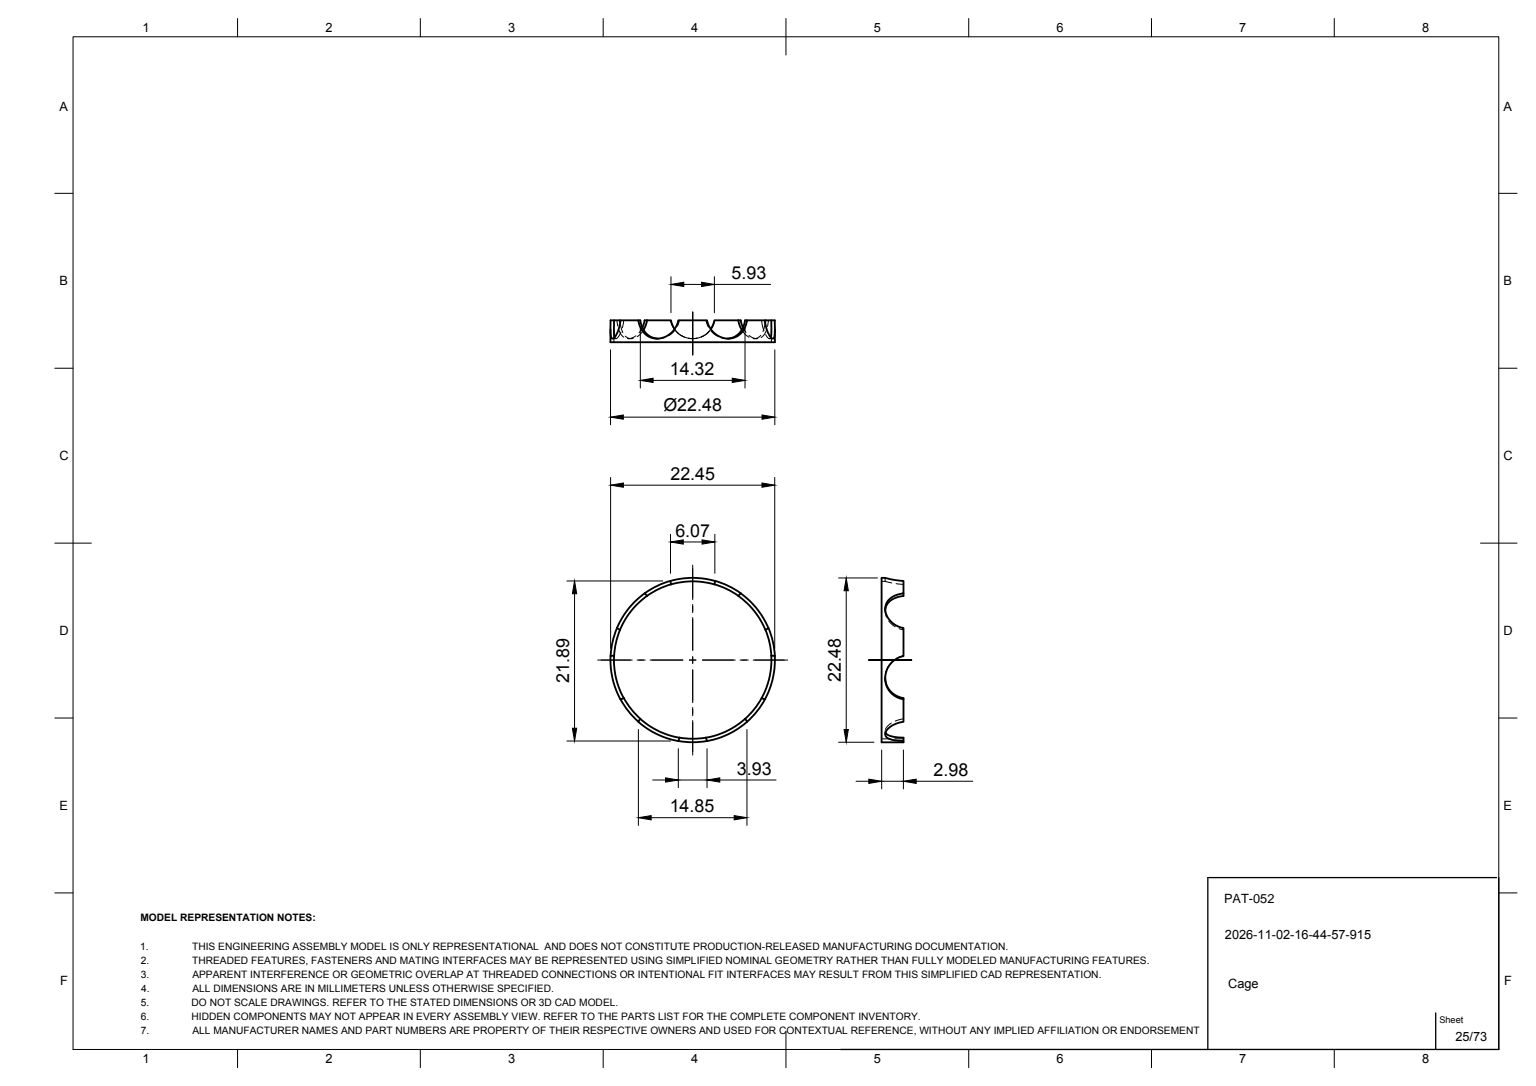
ISO-10303-21;
HEADER;
/* Generated by software containing ST-Developer
 * from STEP Tools, Inc. (www.steptools.com) 
 */

FILE_DESCRIPTION(
/* description */ ('Hand-crank gear train demonstrator'),
/* implementation_level */ '2;1');

FILE_NAME(
/* name */ 'Cage.step',
/* time_stamp */ '2026-10-28T03:22:13-07:00',
/* author */ (''),
/* organization */ (''),
/* preprocessor_version */ 'ST-DEVELOPER v20.2',
/* originating_system */ 'Autodesk Translation Framework v15.17.0.0',
/* authorisation */ '');

FILE_SCHEMA (('AUTOMOTIVE_DESIGN { 1 0 10303 214 3 1 1 }'));
ENDSEC;

DATA;
#10=MECHANICAL_DESIGN_GEOMETRIC_PRESENTATION_REPRESENTATION('',(#1209),#62758);
#859=B_SPLINE_CURVE_WITH_KNOTS('',3,(#24083,#24084,#24085,#24086,#24087,
#24088,#24089,#24090,#24091,#24092,#24093,#24094,#24095,#24096,#24097,#24098,
#24099,#24100,#24101,#24102,#24103,#24104),.UNSPECIFIED.,.F.,.F.,(4,2,2,
2,2,2,2,2,2,2,4),(0.0591825211272536,0.157966726598481,0.236950089897721,
0.315933453196962,0.391576304923761,0.46721915665056,0.54286200837736,0.618504860104159,
0.697488223403399,0.77647158670264,0.875255792173867),.UNSPECIFIED.);
#860=B_SPLINE_CURVE_WITH_KNOTS('',3,(#24108,#24109,#24110,#24111,#24112,
#24113,#24114,#24115,#24116,#24117,#24118,#24119,#24120,#24121,#24122,#24123,
#24124,#24125,#24126,#24127,#24128,#24129),.UNSPECIFIED.,.F.,.F.,(4,2,2,
2,2,2,2,2,2,2,4),(0.0581119756758434,0.106553146291161,0.213106292582322,
0.30849933801665,0.386091982889075,0.4636846277615,0.541277272633925,0.61886991750635,
0.714262962940678,0.820816109231839,0.869257279847157),.UNSPECIFIED.);
#861=B_SPLINE_CURVE_WITH_KNOTS('',3,(#24135,#24136,#24137,#24138,#24139,
#24140,#24141,#24142,#24143,#24144,#24145,#24146,#24147,#24148,#24149,#24150,
#24151,#24152,#24153,#24154,#24155,#24156),.UNSPECIFIED.,.F.,.F.,(4,2,2,
2,2,2,2,2,2,2,4),(0.0581119756758434,0.106553146291161,0.213106292582322,
0.30849933801665,0.386091982889075,0.4636846277615,0.541277272633925,0.61886991750635,
0.714262962940679,0.820816109231839,0.869257279847157),.UNSPECIFIED.);
#862=B_SPLINE_CURVE_WITH_KNOTS('',3,(#24160,#24161,#24162,#24163,#24164,
#24165,#24166,#24167,#24168,#24169,#24170,#24171,#24172,#24173,#24174,#24175,
#24176,#24177,#24178,#24179,#24180,#24181),.UNSPECIFIED.,.F.,.F.,(4,2,2,
2,2,2,2,2,2,2,4),(0.0581119756758433,0.106553146291161,0.213106292582322,
0.308499338016649,0.386091982889075,0.4636846277615,0.541277272633925,0.61886991750635,
0.714262962940678,0.820816109231839,0.869257279847157),.UNSPECIFIED.);
#863=B_SPLINE_CURVE_WITH_KNOTS('',3,(#24190,#24191,#24192,#24193,#24194,
#24195,#24196,#24197,#24198,#24199,#24200,#24201,#24202,#24203,#24204,#24205,
#24206,#24207,#24208,#24209,#24210,#24211),.UNSPECIFIED.,.F.,.F.,(4,2,2,
2,2,2,2,2,2,2,4),(0.0581119756758433,0.106553146291161,0.213106292582322,
0.30849933801665,0.386091982889075,0.4636846277615,0.541277272633925,0.61886991750635,
0.714262962940678,0.820816109231839,0.869257279847157),.UNSPECIFIED.);
#864=B_SPLINE_CURVE_WITH_KNOTS('',3,(#24215,#24216,#24217,#24218,#24219,
#24220,#24221,#24222,#24223,#24224,#24225,#24226,#24227,#24228,#24229,#24230,
#24231,#24232,#24233,#24234,#24235,#24236),.UNSPECIFIED.,.F.,.F.,(4,2,2,
2,2,2,2,2,2,2,4),(0.0581119756758434,0.106553146291161,0.213106292582322,
0.30849933801665,0.386091982889075,0.4636846277615,0.541277272633925,0.61886991750635,
0.714262962940678,0.820816109231839,0.869257279847157),.UNSPECIFIED.);
#865=B_SPLINE_CURVE_WITH_KNOTS('',3,(#24240,#24241,#24242,#24243,#24244,
#24245,#24246,#24247,#24248,#24249,#24250,#24251,#24252,#24253,#24254,#24255,
#24256,#24257,#24258,#24259,#24260,#24261),.UNSPECIFIED.,.F.,.F.,(4,2,2,
2,2,2,2,2,2,2,4),(0.0581119756758434,0.106553146291161,0.213106292582322,
0.30849933801665,0.386091982889075,0.4636846277615,0.541277272633925,0.61886991750635,
0.714262962940678,0.820816109231839,0.869257279847157),.UNSPECIFIED.);
#866=B_SPLINE_CURVE_WITH_KNOTS('',3,(#24265,#24266,#24267,#24268,#24269,
#24270,#24271,#24272,#24273,#24274,#24275,#24276,#24277,#24278,#24279,#24280,
#24281,#24282,#24283,#24284,#24285,#24286),.UNSPECIFIED.,.F.,.F.,(4,2,2,
2,2,2,2,2,2,2,4),(0.0581119756758433,0.106553146291161,0.213106292582322,
0.30849933801665,0.386091982889075,0.4636846277615,0.541277272633925,0.61886991750635,
0.714262962940678,0.820816109231839,0.869257279847157),.UNSPECIFIED.);
#867=B_SPLINE_CURVE_WITH_KNOTS('',3,(#24294,#24295,#24296,#24297,#24298,
#24299,#24300,#24301,#24302,#24303,#24304,#24305,#24306,#24307,#24308,#24309,
#24310,#24311,#24312,#24313,#24314,#24315),.UNSPECIFIED.,.F.,.F.,(4,2,2,
2,2,2,2,2,2,2,4),(0.0591825211272536,0.157966726598481,0.236950089897721,
0.315933453196962,0.391576304923761,0.467219156650561,0.54286200837736,
0.618504860104159,0.697488223403399,0.77647158670264,0.875255792173867),
 .UNSPECIFIED.);
#868=B_SPLINE_CURVE_WITH_KNOTS('',3,(#24323,#24324,#24325,#24326,#24327,
#24328,#24329,#24330,#24331,#24332,#24333,#24334,#24335,#24336,#24337,#24338,
#24339,#24340,#24341,#24342,#24343,#24344),.UNSPECIFIED.,.F.,.F.,(4,2,2,
2,2,2,2,2,2,2,4),(0.0591825211272536,0.157966726598481,0.236950089897722,
0.315933453196962,0.391576304923761,0.467219156650561,0.54286200837736,
0.618504860104159,0.697488223403399,0.77647158670264,0.875255792173867),
 .UNSPECIFIED.);
#869=B_SPLINE_CURVE_WITH_KNOTS('',3,(#24354,#24355,#24356,#24357,#24358,
#24359,#24360,#24361,#24362,#24363,#24364,#24365,#24366,#24367,#24368,#24369,
#24370,#24371,#24372,#24373,#24374,#24375),.UNSPECIFIED.,.F.,.F.,(4,2,2,
2,2,2,2,2,2,2,4),(0.0591825211272536,0.157966726598481,0.236950089897721,
0.315933453196962,0.391576304923761,0.46721915665056,0.54286200837736,0.618504860104159,
0.697488223403399,0.77647158670264,0.875255792173867),.UNSPECIFIED.);
#870=B_SPLINE_CURVE_WITH_KNOTS('',3,(#24383,#24384,#24385,#24386,#24387,
#24388,#24389,#24390,#24391,#24392,#24393,#24394,#24395,#24396,#24397,#24398,
#24399,#24400,#24401,#24402,#24403,#24404),.UNSPECIFIED.,.F.,.F.,(4,2,2,
2,2,2,2,2,2,2,4),(0.0591825211272536,0.157966726598481,0.236950089897721,
0.315933453196962,0.391576304923761,0.46721915665056,0.542862008377359,
0.618504860104159,0.697488223403399,0.776471586702639,0.875255792173867),
 .UNSPECIFIED.);
#871=B_SPLINE_CURVE_WITH_KNOTS('',3,(#24412,#24413,#24414,#24415,#24416,
#24417,#24418,#24419,#24420,#24421,#24422,#24423,#24424,#24425,#24426,#24427,
#24428,#24429,#24430,#24431,#24432,#24433),.UNSPECIFIED.,.F.,.F.,(4,2,2,
2,2,2,2,2,2,2,4),(0.0591825211272536,0.157966726598481,0.236950089897721,
0.315933453196962,0.391576304923761,0.46721915665056,0.54286200837736,0.618504860104159,
0.697488223403399,0.77647158670264,0.875255792173867),.UNSPECIFIED.);
#872=B_SPLINE_CURVE_WITH_KNOTS('',3,(#24442,#24443,#24444,#24445,#24446,
#24447,#24448,#24449,#24450,#24451,#24452,#24453,#24454,#24455,#24456,#24457,
#24458,#24459,#24460,#24461,#24462,#24463),.UNSPECIFIED.,.F.,.F.,(4,2,2,
2,2,2,2,2,2,2,4),(0.0591825211272536,0.157966726598481,0.236950089897721,
0.315933453196962,0.391576304923761,0.46721915665056,0.542862008377359,
0.618504860104159,0.697488223403399,0.776471586702639,0.875255792173867),
 .UNSPECIFIED.);
#998=SPHERICAL_SURFACE('',#17541,0.309556);
#999=SPHERICAL_SURFACE('',#17557,0.309556);
#1000=SPHERICAL_SURFACE('',#17562,0.309556);
#1001=SPHERICAL_SURFACE('',#17568,0.309556);
#1002=SPHERICAL_SURFACE('',#17573,0.309556);
#1003=SPHERICAL_SURFACE('',#17578,0.309556);
#1004=SPHERICAL_SURFACE('',#17586,0.309556);
#1075=SHAPE_REPRESENTATION_RELATIONSHIP('SRR','None',#63048,#1139);
#1139=ADVANCED_BREP_SHAPE_REPRESENTATION('',(#1287),#62702);
#1209=STYLED_ITEM('',(#63462),#1287);
#1287=MANIFOLD_SOLID_BREP('Continuous crown cage',#16390);
#1491=FACE_BOUND('',#3385,.T.);
#1686=PLANE('',#17554);
#1687=PLANE('',#17559);
#1688=PLANE('',#17564);
#1689=PLANE('',#17570);
#1690=PLANE('',#17575);
#1691=PLANE('',#17584);
#1692=PLANE('',#17588);
#1693=PLANE('',#17589);
#2284=FACE_OUTER_BOUND('',#3369,.T.);
#2285=FACE_OUTER_BOUND('',#3370,.T.);
#2286=FACE_OUTER_BOUND('',#3371,.T.);
#2287=FACE_OUTER_BOUND('',#3372,.T.);
#2288=FACE_OUTER_BOUND('',#3373,.T.);
#2289=FACE_OUTER_BOUND('',#3374,.T.);
#2290=FACE_OUTER_BOUND('',#3375,.T.);
#2291=FACE_OUTER_BOUND('',#3376,.T.);
#2292=FACE_OUTER_BOUND('',#3377,.T.);
#2293=FACE_OUTER_BOUND('',#3378,.T.);
#2294=FACE_OUTER_BOUND('',#3379,.T.);
#2295=FACE_OUTER_BOUND('',#3380,.T.);
#2296=FACE_OUTER_BOUND('',#3381,.T.);
#2297=FACE_OUTER_BOUND('',#3382,.T.);
#2298=FACE_OUTER_BOUND('',#3383,.T.);
#2299=FACE_OUTER_BOUND('',#3384,.T.);
#2300=FACE_OUTER_BOUND('',#3386,.T.);
#3369=EDGE_LOOP('',(#11537,#11538,#11539,#11540));
#3370=EDGE_LOOP('',(#11541,#11542,#11543,#11544,#11545,#11546,#11547,#11548,
#11549,#11550,#11551,#11552,#11553,#11554,#11555,#11556,#11557,#11558));
#3371=EDGE_LOOP('',(#11559,#11560,#11561,#11562));
#3372=EDGE_LOOP('',(#11563,#11564,#11565,#11566));
#3373=EDGE_LOOP('',(#11567,#11568,#11569,#11570));
#3374=EDGE_LOOP('',(#11571,#11572,#11573,#11574));
#3375=EDGE_LOOP('',(#11575,#11576,#11577,#11578,#11579,#11580));
#3376=EDGE_LOOP('',(#11581,#11582,#11583,#11584));
#3377=EDGE_LOOP('',(#11585,#11586,#11587,#11588));
#3378=EDGE_LOOP('',(#11589,#11590,#11591,#11592));
#3379=EDGE_LOOP('',(#11593,#11594,#11595,#11596));
#3380=EDGE_LOOP('',(#11597,#11598,#11599,#11600));
#3381=EDGE_LOOP('',(#11601,#11602,#11603,#11604,#11605,#11606,#11607,#11608,
#11609,#11610,#11611,#11612,#11613,#11614,#11615,#11616,#11617,#11618));
#3382=EDGE_LOOP('',(#11619,#11620,#11621,#11622));
#3383=EDGE_LOOP('',(#11623,#11624,#11625,#11626));
#3384=EDGE_LOOP('',(#11627));
#3385=EDGE_LOOP('',(#11628));
#3386=EDGE_LOOP('',(#11629,#11630,#11631,#11632));
#4433=LINE('',#24185,#5565);
#4434=LINE('',#24438,#5566);
#5565=VECTOR('',#19758,1.123812);
#5566=VECTOR('',#19827,1.076188);
#6754=CIRCLE('',#17542,0.303778037777585);
#6755=CIRCLE('',#17543,0.303778037777585);
#6756=CIRCLE('',#17545,1.123812);
#6757=CIRCLE('',#17546,1.123812);
#6758=CIRCLE('',#17547,1.123812);
#6759=CIRCLE('',#17548,1.123812);
#6760=CIRCLE('',#17549,1.123812);
#6761=CIRCLE('',#17550,1.123812);
#6762=CIRCLE('',#17551,1.123812);
#6763=CIRCLE('',#17552,1.123812);
#6764=CIRCLE('',#17553,1.123812);
#6765=CIRCLE('',#17555,1.076188);
#6766=CIRCLE('',#17556,0.303778037777585);
#6767=CIRCLE('',#17558,0.303778037777585);
#6768=CIRCLE('',#17560,1.076188);
#6769=CIRCLE('',#17561,0.303778037777585);
#6770=CIRCLE('',#17563,0.303778037777585);
#6771=CIRCLE('',#17565,1.076188);
#6772=CIRCLE('',#17566,1.076188);
#6773=CIRCLE('',#17567,0.303778037777585);
#6774=CIRCLE('',#17569,0.303778037777585);
#6775=CIRCLE('',#17571,1.076188);
#6776=CIRCLE('',#17572,0.303778037777585);
#6777=CIRCLE('',#17574,0.303778037777585);
#6778=CIRCLE('',#17576,1.076188);
#6779=CIRCLE('',#17577,0.303778037777585);
#6780=CIRCLE('',#17579,0.303778037777585);
#6781=CIRCLE('',#17581,1.076188);
#6782=CIRCLE('',#17582,1.076188);
#6783=CIRCLE('',#17583,1.076188);
#6784=CIRCLE('',#17585,0.303778037777585);
#6785=CIRCLE('',#17587,0.303778037777585);
#7453=VERTEX_POINT('',#24081);
#7454=VERTEX_POINT('',#24082);
#7455=VERTEX_POINT('',#24105);
#7456=VERTEX_POINT('',#24107);
#7457=VERTEX_POINT('',#24132);
#7458=VERTEX_POINT('',#24134);
#7459=VERTEX_POINT('',#24157);
#7460=VERTEX_POINT('',#24159);
#7461=VERTEX_POINT('',#24182);
#7462=VERTEX_POINT('',#24184);
#7463=VERTEX_POINT('',#24187);
#7464=VERTEX_POINT('',#24189);
#7465=VERTEX_POINT('',#24212);
#7466=VERTEX_POINT('',#24214);
#7467=VERTEX_POINT('',#24237);
#7468=VERTEX_POINT('',#24239);
#7469=VERTEX_POINT('',#24262);
#7470=VERTEX_POINT('',#24264);
#7471=VERTEX_POINT('',#24289);
#7472=VERTEX_POINT('',#24293);
#7473=VERTEX_POINT('',#24318);
#7474=VERTEX_POINT('',#24322);
#7475=VERTEX_POINT('',#24347);
#7476=VERTEX_POINT('',#24349);
#7477=VERTEX_POINT('',#24353);
#7478=VERTEX_POINT('',#24378);
#7479=VERTEX_POINT('',#24382);
#7480=VERTEX_POINT('',#24407);
#7481=VERTEX_POINT('',#24411);
#7482=VERTEX_POINT('',#24436);
#7483=VERTEX_POINT('',#24439);
#7484=VERTEX_POINT('',#24441);
#9020=EDGE_CURVE('',#7453,#7454,#859,.T.);
#9021=EDGE_CURVE('',#7455,#7453,#6754,.T.);
#9022=EDGE_CURVE('',#7456,#7455,#860,.T.);
#9023=EDGE_CURVE('',#7454,#7456,#6755,.T.);
#9024=EDGE_CURVE('',#7457,#7455,#6756,.T.);
#9025=EDGE_CURVE('',#7457,#7458,#861,.T.);
#9026=EDGE_CURVE('',#7459,#7458,#6757,.T.);
#9027=EDGE_CURVE('',#7459,#7460,#862,.T.);
#9028=EDGE_CURVE('',#7461,#7460,#6758,.T.);
#9029=EDGE_CURVE('',#7461,#7462,#4433,.T.);
#9030=EDGE_CURVE('',#7462,#7462,#6759,.T.);
#9031=EDGE_CURVE('',#7463,#7461,#6760,.T.);
#9032=EDGE_CURVE('',#7463,#7464,#863,.T.);
#9033=EDGE_CURVE('',#7465,#7464,#6761,.T.);
#9034=EDGE_CURVE('',#7465,#7466,#864,.T.);
#9035=EDGE_CURVE('',#7467,#7466,#6762,.T.);
#9036=EDGE_CURVE('',#7467,#7468,#865,.T.);
#9037=EDGE_CURVE('',#7469,#7468,#6763,.T.);
#9038=EDGE_CURVE('',#7469,#7470,#866,.T.);
#9039=EDGE_CURVE('',#7456,#7470,#6764,.T.);
#9040=EDGE_CURVE('',#7453,#7471,#6765,.T.);
#9041=EDGE_CURVE('',#7471,#7457,#6766,.T.);
#9042=EDGE_CURVE('',#7472,#7471,#867,.T.);
#9043=EDGE_CURVE('',#7458,#7472,#6767,.T.);
#9044=EDGE_CURVE('',#7472,#7473,#6768,.T.);
#9045=EDGE_CURVE('',#7473,#7459,#6769,.T.);
#9046=EDGE_CURVE('',#7474,#7473,#868,.T.);
#9047=EDGE_CURVE('',#7460,#7474,#6770,.T.);
#9048=EDGE_CURVE('',#7474,#7475,#6771,.T.);
#9049=EDGE_CURVE('',#7475,#7476,#6772,.T.);
#9050=EDGE_CURVE('',#7476,#7463,#6773,.T.);
#9051=EDGE_CURVE('',#7477,#7476,#869,.T.);
#9052=EDGE_CURVE('',#7464,#7477,#6774,.T.);
#9053=EDGE_CURVE('',#7477,#7478,#6775,.T.);
#9054=EDGE_CURVE('',#7478,#7465,#6776,.T.);
#9055=EDGE_CURVE('',#7479,#7478,#870,.T.);
#9056=EDGE_CURVE('',#7466,#7479,#6777,.T.);
#9057=EDGE_CURVE('',#7479,#7480,#6778,.T.);
#9058=EDGE_CURVE('',#7480,#7467,#6779,.T.);
#9059=EDGE_CURVE('',#7481,#7480,#871,.T.);
#9060=EDGE_CURVE('',#7468,#7481,#6780,.T.);
#9061=EDGE_CURVE('',#7482,#7482,#6781,.T.);
#9062=EDGE_CURVE('',#7482,#7475,#4434,.T.);
#9063=EDGE_CURVE('',#7483,#7454,#6782,.T.);
#9064=EDGE_CURVE('',#7483,#7484,#872,.T.);
#9065=EDGE_CURVE('',#7481,#7484,#6783,.T.);
#9066=EDGE_CURVE('',#7470,#7483,#6784,.T.);
#9067=EDGE_CURVE('',#7484,#7469,#6785,.T.);
#11537=ORIENTED_EDGE('',*,*,#9020,.F.);
#11538=ORIENTED_EDGE('',*,*,#9021,.F.);
#11539=ORIENTED_EDGE('',*,*,#9022,.F.);
#11540=ORIENTED_EDGE('',*,*,#9023,.F.);
#11541=ORIENTED_EDGE('',*,*,#9022,.T.);
#11542=ORIENTED_EDGE('',*,*,#9024,.F.);
#11543=ORIENTED_EDGE('',*,*,#9025,.T.);
#11544=ORIENTED_EDGE('',*,*,#9026,.F.);
#11545=ORIENTED_EDGE('',*,*,#9027,.T.);
#11546=ORIENTED_EDGE('',*,*,#9028,.F.);
#11547=ORIENTED_EDGE('',*,*,#9029,.T.);
#11548=ORIENTED_EDGE('',*,*,#9030,.F.);
#11549=ORIENTED_EDGE('',*,*,#9029,.F.);
#11550=ORIENTED_EDGE('',*,*,#9031,.F.);
#11551=ORIENTED_EDGE('',*,*,#9032,.T.);
#11552=ORIENTED_EDGE('',*,*,#9033,.F.);
#11553=ORIENTED_EDGE('',*,*,#9034,.T.);
#11554=ORIENTED_EDGE('',*,*,#9035,.F.);
#11555=ORIENTED_EDGE('',*,*,#9036,.T.);
#11556=ORIENTED_EDGE('',*,*,#9037,.F.);
#11557=ORIENTED_EDGE('',*,*,#9038,.T.);
#11558=ORIENTED_EDGE('',*,*,#9039,.F.);
#11559=ORIENTED_EDGE('',*,*,#9021,.T.);
#11560=ORIENTED_EDGE('',*,*,#9040,.T.);
#11561=ORIENTED_EDGE('',*,*,#9041,.T.);
#11562=ORIENTED_EDGE('',*,*,#9024,.T.);
#11563=ORIENTED_EDGE('',*,*,#9042,.F.);
#11564=ORIENTED_EDGE('',*,*,#9043,.F.);
#11565=ORIENTED_EDGE('',*,*,#9025,.F.);
#11566=ORIENTED_EDGE('',*,*,#9041,.F.);
#11567=ORIENTED_EDGE('',*,*,#9043,.T.);
#11568=ORIENTED_EDGE('',*,*,#9044,.T.);
#11569=ORIENTED_EDGE('',*,*,#9045,.T.);
#11570=ORIENTED_EDGE('',*,*,#9026,.T.);
#11571=ORIENTED_EDGE('',*,*,#9046,.F.);
#11572=ORIENTED_EDGE('',*,*,#9047,.F.);
#11573=ORIENTED_EDGE('',*,*,#9027,.F.);
#11574=ORIENTED_EDGE('',*,*,#9045,.F.);
#11575=ORIENTED_EDGE('',*,*,#9047,.T.);
#11576=ORIENTED_EDGE('',*,*,#9048,.T.);
#11577=ORIENTED_EDGE('',*,*,#9049,.T.);
#11578=ORIENTED_EDGE('',*,*,#9050,.T.);
#11579=ORIENTED_EDGE('',*,*,#9031,.T.);
#11580=ORIENTED_EDGE('',*,*,#9028,.T.);
#11581=ORIENTED_EDGE('',*,*,#9051,.F.);
#11582=ORIENTED_EDGE('',*,*,#9052,.F.);
#11583=ORIENTED_EDGE('',*,*,#9032,.F.);
#11584=ORIENTED_EDGE('',*,*,#9050,.F.);
#11585=ORIENTED_EDGE('',*,*,#9052,.T.);
#11586=ORIENTED_EDGE('',*,*,#9053,.T.);
#11587=ORIENTED_EDGE('',*,*,#9054,.T.);
#11588=ORIENTED_EDGE('',*,*,#9033,.T.);
#11589=ORIENTED_EDGE('',*,*,#9055,.F.);
#11590=ORIENTED_EDGE('',*,*,#9056,.F.);
#11591=ORIENTED_EDGE('',*,*,#9034,.F.);
#11592=ORIENTED_EDGE('',*,*,#9054,.F.);
#11593=ORIENTED_EDGE('',*,*,#9056,.T.);
#11594=ORIENTED_EDGE('',*,*,#9057,.T.);
#11595=ORIENTED_EDGE('',*,*,#9058,.T.);
#11596=ORIENTED_EDGE('',*,*,#9035,.T.);
#11597=ORIENTED_EDGE('',*,*,#9036,.F.);
#11598=ORIENTED_EDGE('',*,*,#9058,.F.);
#11599=ORIENTED_EDGE('',*,*,#9059,.F.);
#11600=ORIENTED_EDGE('',*,*,#9060,.F.);
#11601=ORIENTED_EDGE('',*,*,#9061,.F.);
#11602=ORIENTED_EDGE('',*,*,#9062,.T.);
#11603=ORIENTED_EDGE('',*,*,#9048,.F.);
#11604=ORIENTED_EDGE('',*,*,#9046,.T.);
#11605=ORIENTED_EDGE('',*,*,#9044,.F.);
#11606=ORIENTED_EDGE('',*,*,#9042,.T.);
#11607=ORIENTED_EDGE('',*,*,#9040,.F.);
#11608=ORIENTED_EDGE('',*,*,#9020,.T.);
#11609=ORIENTED_EDGE('',*,*,#9063,.F.);
#11610=ORIENTED_EDGE('',*,*,#9064,.T.);
#11611=ORIENTED_EDGE('',*,*,#9065,.F.);
#11612=ORIENTED_EDGE('',*,*,#9059,.T.);
#11613=ORIENTED_EDGE('',*,*,#9057,.F.);
#11614=ORIENTED_EDGE('',*,*,#9055,.T.);
#11615=ORIENTED_EDGE('',*,*,#9053,.F.);
#11616=ORIENTED_EDGE('',*,*,#9051,.T.);
#11617=ORIENTED_EDGE('',*,*,#9049,.F.);
#11618=ORIENTED_EDGE('',*,*,#9062,.F.);
#11619=ORIENTED_EDGE('',*,*,#9023,.T.);
#11620=ORIENTED_EDGE('',*,*,#9039,.T.);
#11621=ORIENTED_EDGE('',*,*,#9066,.T.);
#11622=ORIENTED_EDGE('',*,*,#9063,.T.);
#11623=ORIENTED_EDGE('',*,*,#9038,.F.);
#11624=ORIENTED_EDGE('',*,*,#9067,.F.);
#11625=ORIENTED_EDGE('',*,*,#9064,.F.);
#11626=ORIENTED_EDGE('',*,*,#9066,.F.);
#11627=ORIENTED_EDGE('',*,*,#9030,.T.);
#11628=ORIENTED_EDGE('',*,*,#9061,.T.);
#11629=ORIENTED_EDGE('',*,*,#9060,.T.);
#11630=ORIENTED_EDGE('',*,*,#9065,.T.);
#11631=ORIENTED_EDGE('',*,*,#9067,.T.);
#11632=ORIENTED_EDGE('',*,*,#9037,.T.);
#15259=CYLINDRICAL_SURFACE('',#17544,1.123812);
#15260=CYLINDRICAL_SURFACE('',#17580,1.076188);
#15594=ADVANCED_FACE('',(#2284),#998,.F.);
#15595=ADVANCED_FACE('',(#2285),#15259,.T.);
#15596=ADVANCED_FACE('',(#2286),#1686,.T.);
#15597=ADVANCED_FACE('',(#2287),#999,.F.);
#15598=ADVANCED_FACE('',(#2288),#1687,.T.);
#15599=ADVANCED_FACE('',(#2289),#1000,.F.);
#15600=ADVANCED_FACE('',(#2290),#1688,.T.);
#15601=ADVANCED_FACE('',(#2291),#1001,.F.);
#15602=ADVANCED_FACE('',(#2292),#1689,.T.);
#15603=ADVANCED_FACE('',(#2293),#1002,.F.);
#15604=ADVANCED_FACE('',(#2294),#1690,.T.);
#15605=ADVANCED_FACE('',(#2295),#1003,.F.);
#15606=ADVANCED_FACE('',(#2296),#15260,.F.);
#15607=ADVANCED_FACE('',(#2297),#1691,.T.);
#15608=ADVANCED_FACE('',(#2298),#1004,.F.);
#15609=ADVANCED_FACE('',(#2299,#1491),#1692,.T.);
#15610=ADVANCED_FACE('',(#2300),#1693,.T.);
#16390=CLOSED_SHELL('',(#15594,#15595,#15596,#15597,#15598,#15599,#15600,
#15601,#15602,#15603,#15604,#15605,#15606,#15607,#15608,#15609,#15610));
#17540=AXIS2_PLACEMENT_3D('',#24079,#19742,#19743);
#17541=AXIS2_PLACEMENT_3D('',#24080,#19744,#19745);
#17542=AXIS2_PLACEMENT_3D('',#24106,#19746,#19747);
#17543=AXIS2_PLACEMENT_3D('',#24130,#19748,#19749);
#17544=AXIS2_PLACEMENT_3D('',#24131,#19750,#19751);
#17545=AXIS2_PLACEMENT_3D('',#24133,#19752,#19753);
#17546=AXIS2_PLACEMENT_3D('',#24158,#19754,#19755);
#17547=AXIS2_PLACEMENT_3D('',#24183,#19756,#19757);
#17548=AXIS2_PLACEMENT_3D('',#24186,#19759,#19760);
#17549=AXIS2_PLACEMENT_3D('',#24188,#19761,#19762);
#17550=AXIS2_PLACEMENT_3D('',#24213,#19763,#19764);
#17551=AXIS2_PLACEMENT_3D('',#24238,#19765,#19766);
#17552=AXIS2_PLACEMENT_3D('',#24263,#19767,#19768);
#17553=AXIS2_PLACEMENT_3D('',#24287,#19769,#19770);
#17554=AXIS2_PLACEMENT_3D('',#24288,#19771,#19772);
#17555=AXIS2_PLACEMENT_3D('',#24290,#19773,#19774);
#17556=AXIS2_PLACEMENT_3D('',#24291,#19775,#19776);
#17557=AXIS2_PLACEMENT_3D('',#24292,#19777,#19778);
#17558=AXIS2_PLACEMENT_3D('',#24316,#19779,#19780);
#17559=AXIS2_PLACEMENT_3D('',#24317,#19781,#19782);
#17560=AXIS2_PLACEMENT_3D('',#24319,#19783,#19784);
#17561=AXIS2_PLACEMENT_3D('',#24320,#19785,#19786);
#17562=AXIS2_PLACEMENT_3D('',#24321,#19787,#19788);
#17563=AXIS2_PLACEMENT_3D('',#24345,#19789,#19790);
#17564=AXIS2_PLACEMENT_3D('',#24346,#19791,#19792);
#17565=AXIS2_PLACEMENT_3D('',#24348,#19793,#19794);
#17566=AXIS2_PLACEMENT_3D('',#24350,#19795,#19796);
#17567=AXIS2_PLACEMENT_3D('',#24351,#19797,#19798);
#17568=AXIS2_PLACEMENT_3D('',#24352,#19799,#19800);
#17569=AXIS2_PLACEMENT_3D('',#24376,#19801,#19802);
#17570=AXIS2_PLACEMENT_3D('',#24377,#19803,#19804);
#17571=AXIS2_PLACEMENT_3D('',#24379,#19805,#19806);
#17572=AXIS2_PLACEMENT_3D('',#24380,#19807,#19808);
#17573=AXIS2_PLACEMENT_3D('',#24381,#19809,#19810);
#17574=AXIS2_PLACEMENT_3D('',#24405,#19811,#19812);
#17575=AXIS2_PLACEMENT_3D('',#24406,#19813,#19814);
#17576=AXIS2_PLACEMENT_3D('',#24408,#19815,#19816);
#17577=AXIS2_PLACEMENT_3D('',#24409,#19817,#19818);
#17578=AXIS2_PLACEMENT_3D('',#24410,#19819,#19820);
#17579=AXIS2_PLACEMENT_3D('',#24434,#19821,#19822);
#17580=AXIS2_PLACEMENT_3D('',#24435,#19823,#19824);
#17581=AXIS2_PLACEMENT_3D('',#24437,#19825,#19826);
#17582=AXIS2_PLACEMENT_3D('',#24440,#19828,#19829);
#17583=AXIS2_PLACEMENT_3D('',#24464,#19830,#19831);
#17584=AXIS2_PLACEMENT_3D('',#24465,#19832,#19833);
#17585=AXIS2_PLACEMENT_3D('',#24466,#19834,#19835);
#17586=AXIS2_PLACEMENT_3D('',#24467,#19836,#19837);
#17587=AXIS2_PLACEMENT_3D('',#24468,#19838,#19839);
#17588=AXIS2_PLACEMENT_3D('',#24469,#19840,#19841);
#17589=AXIS2_PLACEMENT_3D('',#24470,#19842,#19843);
#19742=DIRECTION('axis',(0.,0.,1.));
#19743=DIRECTION('refdir',(1.,0.,0.));
#19744=DIRECTION('center_axis',(0.,0.,1.));
#19745=DIRECTION('ref_axis',(1.,0.,0.));
#19746=DIRECTION('center_axis',(0.,-1.,0.));
#19747=DIRECTION('ref_axis',(0.,0.,-1.));
#19748=DIRECTION('center_axis',(0.,-1.,0.));
#19749=DIRECTION('ref_axis',(0.,0.,-1.));
#19750=DIRECTION('center_axis',(0.,1.,0.));
#19751=DIRECTION('ref_axis',(1.,0.,0.));
#19752=DIRECTION('center_axis',(0.,1.,0.));
#19753=DIRECTION('ref_axis',(1.,0.,0.));
#19754=DIRECTION('center_axis',(0.,1.,0.));
#19755=DIRECTION('ref_axis',(1.,0.,0.));
#19756=DIRECTION('center_axis',(0.,1.,0.));
#19757=DIRECTION('ref_axis',(1.,0.,0.));
#19758=DIRECTION('',(0.,-1.,0.));
#19759=DIRECTION('center_axis',(0.,-1.,0.));
#19760=DIRECTION('ref_axis',(1.,0.,0.));
#19761=DIRECTION('center_axis',(0.,1.,0.));
#19762=DIRECTION('ref_axis',(1.,0.,0.));
#19763=DIRECTION('center_axis',(0.,1.,0.));
#19764=DIRECTION('ref_axis',(1.,0.,0.));
#19765=DIRECTION('center_axis',(0.,1.,0.));
#19766=DIRECTION('ref_axis',(1.,0.,0.));
#19767=DIRECTION('center_axis',(0.,1.,0.));
#19768=DIRECTION('ref_axis',(1.,0.,0.));
#19769=DIRECTION('center_axis',(0.,1.,0.));
#19770=DIRECTION('ref_axis',(1.,0.,0.));
#19771=DIRECTION('center_axis',(0.,1.,0.));
#19772=DIRECTION('ref_axis',(1.,0.,0.));
#19773=DIRECTION('center_axis',(0.,-1.,0.));
#19774=DIRECTION('ref_axis',(1.,0.,0.));
#19775=DIRECTION('center_axis',(0.,-1.,0.));
#19776=DIRECTION('ref_axis',(0.,0.,-1.));
#19777=DIRECTION('center_axis',(8.96625347776458E-17,0.,1.));
#19778=DIRECTION('ref_axis',(1.,0.,0.));
#19779=DIRECTION('center_axis',(0.,-1.,0.));
#19780=DIRECTION('ref_axis',(0.,0.,-1.));
#19781=DIRECTION('center_axis',(0.,1.,0.));
#19782=DIRECTION('ref_axis',(1.,0.,0.));
#19783=DIRECTION('center_axis',(0.,-1.,0.));
#19784=DIRECTION('ref_axis',(1.,0.,0.));
#19785=DIRECTION('center_axis',(0.,-1.,0.));
#19786=DIRECTION('ref_axis',(0.,0.,-1.));
#19787=DIRECTION('center_axis',(0.,0.,1.));
#19788=DIRECTION('ref_axis',(1.,0.,0.));
#19789=DIRECTION('center_axis',(0.,-1.,0.));
#19790=DIRECTION('ref_axis',(0.,0.,-1.));
#19791=DIRECTION('center_axis',(0.,1.,0.));
#19792=DIRECTION('ref_axis',(1.,0.,0.));
#19793=DIRECTION('center_axis',(0.,-1.,0.));
#19794=DIRECTION('ref_axis',(1.,0.,0.));
#19795=DIRECTION('center_axis',(0.,-1.,0.));
#19796=DIRECTION('ref_axis',(1.,0.,0.));
#19797=DIRECTION('center_axis',(0.,-1.,0.));
#19798=DIRECTION('ref_axis',(0.,0.,-1.));
#19799=DIRECTION('center_axis',(0.,0.,1.));
#19800=DIRECTION('ref_axis',(1.,0.,0.));
#19801=DIRECTION('center_axis',(0.,-1.,0.));
#19802=DIRECTION('ref_axis',(0.,0.,-1.));
#19803=DIRECTION('center_axis',(0.,1.,0.));
#19804=DIRECTION('ref_axis',(1.,0.,0.));
#19805=DIRECTION('center_axis',(0.,-1.,0.));
#19806=DIRECTION('ref_axis',(1.,0.,0.));
#19807=DIRECTION('center_axis',(0.,-1.,0.));
#19808=DIRECTION('ref_axis',(0.,0.,-1.));
#19809=DIRECTION('center_axis',(8.96625347776458E-17,0.,1.));
#19810=DIRECTION('ref_axis',(1.,0.,0.));
#19811=DIRECTION('center_axis',(0.,-1.,0.));
#19812=DIRECTION('ref_axis',(0.,0.,-1.));
#19813=DIRECTION('center_axis',(0.,1.,0.));
#19814=DIRECTION('ref_axis',(1.,0.,0.));
#19815=DIRECTION('center_axis',(0.,-1.,0.));
#19816=DIRECTION('ref_axis',(1.,0.,0.));
#19817=DIRECTION('center_axis',(0.,-1.,0.));
#19818=DIRECTION('ref_axis',(0.,0.,-1.));
#19819=DIRECTION('center_axis',(0.,0.,1.));
#19820=DIRECTION('ref_axis',(1.,0.,0.));
#19821=DIRECTION('center_axis',(0.,-1.,0.));
#19822=DIRECTION('ref_axis',(0.,0.,-1.));
#19823=DIRECTION('center_axis',(0.,1.,0.));
#19824=DIRECTION('ref_axis',(1.,0.,0.));
#19825=DIRECTION('center_axis',(0.,1.,0.));
#19826=DIRECTION('ref_axis',(1.,0.,0.));
#19827=DIRECTION('',(0.,1.,0.));
#19828=DIRECTION('center_axis',(0.,-1.,0.));
#19829=DIRECTION('ref_axis',(1.,0.,0.));
#19830=DIRECTION('center_axis',(0.,-1.,0.));
#19831=DIRECTION('ref_axis',(1.,0.,0.));
#19832=DIRECTION('center_axis',(0.,1.,0.));
#19833=DIRECTION('ref_axis',(1.,0.,0.));
#19834=DIRECTION('center_axis',(0.,-1.,0.));
#19835=DIRECTION('ref_axis',(0.,0.,-1.));
#19836=DIRECTION('center_axis',(0.,0.,1.));
#19837=DIRECTION('ref_axis',(1.,0.,0.));
#19838=DIRECTION('center_axis',(0.,-1.,0.));
#19839=DIRECTION('ref_axis',(0.,0.,-1.));
#19840=DIRECTION('center_axis',(0.,-1.,0.));
#19841=DIRECTION('ref_axis',(-1.,0.,0.));
#19842=DIRECTION('center_axis',(0.,1.,0.));
#19843=DIRECTION('ref_axis',(1.,0.,0.));
#24079=CARTESIAN_POINT('',(0.,0.,0.));
#24080=CARTESIAN_POINT('Origin',(0.685838782044607,0.,0.860014630714833));
#24081=CARTESIAN_POINT('',(0.413083465285518,-0.05953,0.993751811093549));
#24082=CARTESIAN_POINT('',(0.876916659919095,-0.05953,0.623857181492959));
#24083=CARTESIAN_POINT('Ctrl Pts',(0.413083465285518,-0.05953,0.993751811093549));
#24084=CARTESIAN_POINT('Ctrl Pts',(0.419070565453383,-0.0925528133349865,
0.991263089003441));
#24085=CARTESIAN_POINT('Ctrl Pts',(0.430199341854858,-0.124911173756694,
0.986608710139579));
#24086=CARTESIAN_POINT('Ctrl Pts',(0.457978755888596,-0.177924977804098,
0.973971221090534));
#24087=CARTESIAN_POINT('Ctrl Pts',(0.473077587363685,-0.199697230012983,
0.966820759530997));
#24088=CARTESIAN_POINT('Ctrl Pts',(0.507057380724533,-0.237895043532788,
0.949440676105255));
#24089=CARTESIAN_POINT('Ctrl Pts',(0.525933334162555,-0.254319232363049,
0.939198248544428));
#24090=CARTESIAN_POINT('Ctrl Pts',(0.564362943424238,-0.28018331644634,
0.916597376014514));
#24091=CARTESIAN_POINT('Ctrl Pts',(0.585840553788742,-0.29104845371857,
0.903141581680914));
#24092=CARTESIAN_POINT('Ctrl Pts',(0.629305439856167,-0.30527573347708,
0.873412008702649));
#24093=CARTESIAN_POINT('Ctrl Pts',(0.651278921914856,-0.308638795020976,
0.857118508332695));
#24094=CARTESIAN_POINT('Ctrl Pts',(0.690705563850638,-0.308638795020976,
0.825676810575914));
#24095=CARTESIAN_POINT('Ctrl Pts',(0.711480111898423,-0.30527573347708,
0.807879894508811));
#24096=CARTESIAN_POINT('Ctrl Pts',(0.750136149454208,-0.29104845371857,
0.772120216227122));
#24097=CARTESIAN_POINT('Ctrl Pts',(0.768033796848072,-0.28018331644634,
0.754175290318038));
#24098=CARTESIAN_POINT('Ctrl Pts',(0.798619410861634,-0.254319232363049,
0.721738358858166));
#24099=CARTESIAN_POINT('Ctrl Pts',(0.812805334167529,-0.237895043532788,
0.705614819529209));
#24100=CARTESIAN_POINT('Ctrl Pts',(0.837310877969633,-0.199697230012983,
0.676354402927683));
#24101=CARTESIAN_POINT('Ctrl Pts',(0.847641868610495,-0.177924977804098,
0.663225258065736));
#24102=CARTESIAN_POINT('Ctrl Pts',(0.866144010579847,-0.124911173756694,
0.638954437806245));
#24103=CARTESIAN_POINT('Ctrl Pts',(0.873158080166742,-0.0925528133349865,
0.62914037979579));
#24104=CARTESIAN_POINT('Ctrl Pts',(0.876916659919095,-0.05953,0.623857181492959));
#24105=CARTESIAN_POINT('',(0.437601487681057,-0.05953,1.03511272300331));
#24106=CARTESIAN_POINT('Origin',(0.685838782044607,-0.05953,0.860014630714833));
#24107=CARTESIAN_POINT('',(0.911784794170997,-0.05953,0.656964154625313));
#24108=CARTESIAN_POINT('Ctrl Pts',(0.911784794170998,-0.0595300000000001,
0.656964154625312));
#24109=CARTESIAN_POINT('Ctrl Pts',(0.909827729890942,-0.0762225747374255,
0.659680317203144));
#24110=CARTESIAN_POINT('Ctrl Pts',(0.907004864562642,-0.0928409665394228,
0.663576540841106));
#24111=CARTESIAN_POINT('Ctrl Pts',(0.895234408667242,-0.144299303100741,
0.679480524217551));
#24112=CARTESIAN_POINT('Ctrl Pts',(0.882797231409153,-0.177024326825049,
0.695831250979106));
#24113=CARTESIAN_POINT('Ctrl Pts',(0.854332839576145,-0.227269801620064,
0.73042219438957));
#24114=CARTESIAN_POINT('Ctrl Pts',(0.834863020612702,-0.251265615809407,
0.752807465209441));
#24115=CARTESIAN_POINT('Ctrl Pts',(0.800439809856111,-0.279889827963178,
0.789147407129766));
#24116=CARTESIAN_POINT('Ctrl Pts',(0.781998747691871,-0.290879136862659,
0.80756613568454));
#24117=CARTESIAN_POINT('Ctrl Pts',(0.742239891936898,-0.305251990234487,
0.844254137480382));
#24118=CARTESIAN_POINT('Ctrl Pts',(0.720906778729541,-0.308638795020976,
0.862505527716294));
#24119=CARTESIAN_POINT('Ctrl Pts',(0.680463863683392,-0.308638795020976,
0.894757676234429));
#24120=CARTESIAN_POINT('Ctrl Pts',(0.657923009631182,-0.305251990234488,
0.91149460735272));
#24121=CARTESIAN_POINT('Ctrl Pts',(0.613307674922609,-0.290879136862659,
0.942092777160053));
#24122=CARTESIAN_POINT('Ctrl Pts',(0.591247219971725,-0.279889827963178,
0.955972930713954));
#24123=CARTESIAN_POINT('Ctrl Pts',(0.548158511259202,-0.251265615809407,
0.981446681891443));
#24124=CARTESIAN_POINT('Ctrl Pts',(0.522002043615455,-0.227269801620063,
0.995447160474328));
#24125=CARTESIAN_POINT('Ctrl Pts',(0.481944444320713,-0.177024326825049,
1.01550068154148));
#24126=CARTESIAN_POINT('Ctrl Pts',(0.463236132117164,-0.14429930310074,
1.0239876538093));
#24127=CARTESIAN_POINT('Ctrl Pts',(0.445111721969657,-0.0928409665394226,
1.03192403056628));
#24128=CARTESIAN_POINT('Ctrl Pts',(0.440685038163619,-0.0762225747374254,
1.03380912944435));
#24129=CARTESIAN_POINT('Ctrl Pts',(0.437601487681056,-0.05953,1.03511272300331));
#24130=CARTESIAN_POINT('Origin',(0.685838782044607,-0.05953,0.860014630714833));
#24131=CARTESIAN_POINT('Origin',(0.,-0.208355,0.));
#24132=CARTESIAN_POINT('',(0.0548532617164168,-0.05953,1.12247250791415));
#24133=CARTESIAN_POINT('Origin',(0.,-0.05953,0.));
#24134=CARTESIAN_POINT('',(-0.536443649899848,-0.05953,0.987512846410683));
#24135=CARTESIAN_POINT('Ctrl Pts',(0.0548532617164173,-0.0595300000000001,
1.12247250791414));
#24136=CARTESIAN_POINT('Ctrl Pts',(0.05150947068137,-0.0762225747374254,
1.12263591311425));
#24137=CARTESIAN_POINT('Ctrl Pts',(0.0467032526342597,-0.0928409665394227,
1.12285816383385));
#24138=CARTESIAN_POINT('Ctrl Pts',(0.0269302585198975,-0.144299303100741,
1.12357162229597));
#24139=CARTESIAN_POINT('Ctrl Pts',(0.006392292392153,-0.177024326825049,
1.12404235695137));
#24140=CARTESIAN_POINT('Ctrl Pts',(-0.0383992541984087,-0.227269801620063,
1.12335509974011));
#24141=CARTESIAN_POINT('Ctrl Pts',(-0.0680399972366993,-0.251265615809407,
1.12208997038458));
#24142=CARTESIAN_POINT('Ctrl Pts',(-0.117914228755037,-0.279889827963178,
1.1178344036749));
#24143=CARTESIAN_POINT('Ctrl Pts',(-0.14381238480104,-0.290879136862659,
1.11490049012186));
#24144=CARTESIAN_POINT('Ctrl Pts',(-0.19728546073067,-0.305251990234488,
1.10669035995599));
#24145=CARTESIAN_POINT('Ctrl Pts',(-0.224855950742601,-0.308638795020976,
1.10139101611326));
#24146=CARTESIAN_POINT('Ctrl Pts',(-0.275287440920027,-0.308638795020976,
1.0898803575765));
#24147=CARTESIAN_POINT('Ctrl Pts',(-0.302426893214945,-0.305251990234488,
1.08269251410343));
#24148=CARTESIAN_POINT('Ctrl Pts',(-0.35416671187353,-0.290879136862659,
1.06688848765783));
#24149=CARTESIAN_POINT('Ctrl Pts',(-0.3787731215897,-0.279889827963178,
1.05829506364875));
#24150=CARTESIAN_POINT('Ctrl Pts',(-0.425554672694338,-0.251265615809407,
1.04048957871266));
#24151=CARTESIAN_POINT('Ctrl Pts',(-0.452808978448581,-0.227269801620063,
1.02876878445619));
#24152=CARTESIAN_POINT('Ctrl Pts',(-0.493462957200432,-0.177024326825049,
1.0099536580922));
#24153=CARTESIAN_POINT('Ctrl Pts',(-0.511762781179148,-0.14429930310074,
1.00061845128527));
#24154=CARTESIAN_POINT('Ctrl Pts',(-0.529268075276157,-0.0928409665394226,
0.991396466802468));
#24155=CARTESIAN_POINT('Ctrl Pts',(-0.533501897135713,-0.0762225747374254,
0.989110885965947));
#24156=CARTESIAN_POINT('Ctrl Pts',(-0.536443649899848,-0.0595300000000001,
0.987512846410683));
#24157=CARTESIAN_POINT('',(-0.843383895613249,-0.05953,0.742736168477219));
#24158=CARTESIAN_POINT('Origin',(0.,-0.05953,0.));
#24159=CARTESIAN_POINT('',(-1.10653577764992,-0.05953,0.196295654879792));
#24160=CARTESIAN_POINT('Ctrl Pts',(-0.843383895613249,-0.0595300000000001,
0.742736168477219));
#24161=CARTESIAN_POINT('Ctrl Pts',(-0.84559647055299,-0.0762225747374255,
0.740223768851062));
#24162=CARTESIAN_POINT('Ctrl Pts',(-0.848766861100456,-0.0928409665394227,
0.736604687327351));
#24163=CARTESIAN_POINT('Ctrl Pts',(-0.861652925570091,-0.144299303100741,
0.721590372101268));
#24164=CARTESIAN_POINT('Ctrl Pts',(-0.87482617317514,-0.177024326825049,
0.705826641853758));
#24165=CARTESIAN_POINT('Ctrl Pts',(-0.902215926359523,-0.227269801620063,
0.670378702718353));
#24166=CARTESIAN_POINT('Ctrl Pts',(-0.919707509403859,-0.251265615809407,
0.646415841396062));
#24167=CARTESIAN_POINT('Ctrl Pts',(-0.947476448101718,-0.279889827963178,
0.604769294586516));
#24168=CARTESIAN_POINT('Ctrl Pts',(-0.961329858300736,-0.290879136862659,
0.582692035672022));
#24169=CARTESIAN_POINT('Ctrl Pts',(-0.988250837578047,-0.305251990234488,
0.535766169015486));
#24170=CARTESIAN_POINT('Ctrl Pts',(-1.00129756308006,-0.308638795020976,
0.510906605094603));
#24171=CARTESIAN_POINT('Ctrl Pts',(-1.02374168767024,-0.308638795020976,
0.46430090015576));
#24172=CARTESIAN_POINT('Ctrl Pts',(-1.03504317708586,-0.305251990234488,
0.438600874831839));
#24173=CARTESIAN_POINT('Ctrl Pts',(-1.05494634094458,-0.290879136862659,
0.388295406390235));
#24174=CARTESIAN_POINT('Ctrl Pts',(-1.06356957703048,-0.279889827963178,
0.363699428370917));
#24175=CARTESIAN_POINT('Ctrl Pts',(-1.0788165083757,-0.251265615809407,
0.316022600643821));
#24176=CARTESIAN_POINT('Ctrl Pts',(-1.08664560412098,-0.227269801620063,
0.287406530683752));
#24177=CARTESIAN_POINT('Ctrl Pts',(-1.09728268713976,-0.177024326825049,
0.243890930799337));
#24178=CARTESIAN_POINT('Ctrl Pts',(-1.10139388218929,-0.144299303100741,
0.22376314604679));
#24179=CARTESIAN_POINT('Ctrl Pts',(-1.10509821673782,-0.0928409665394227,
0.204327142733961));
#24180=CARTESIAN_POINT('Ctrl Pts',(-1.10595102243643,-0.0762225747374254,
0.199591971170104));
#24181=CARTESIAN_POINT('Ctrl Pts',(-1.10653577764992,-0.0595300000000001,
0.196295654879792));
#24182=CARTESIAN_POINT('',(-1.123812,-0.05953,1.37627276864339E-16));
#24183=CARTESIAN_POINT('Origin',(0.,-0.05953,0.));
#24184=CARTESIAN_POINT('',(-1.123812,-0.35718,1.37627276864339E-16));
#24185=CARTESIAN_POINT('',(-1.123812,-0.208355,1.37627276864339E-16));
#24186=CARTESIAN_POINT('Origin',(0.,-0.35718,0.));
#24187=CARTESIAN_POINT('',(-1.10653577764992,-0.05953,-0.196295654879793));
#24188=CARTESIAN_POINT('Origin',(0.,-0.05953,0.));
#24189=CARTESIAN_POINT('',(-0.843383895613249,-0.05953,-0.742736168477219));
#24190=CARTESIAN_POINT('Ctrl Pts',(-1.10653577764992,-0.0595300000000001,
-0.196295654879792));
#24191=CARTESIAN_POINT('Ctrl Pts',(-1.10595102243643,-0.0762225747374255,
-0.199591971170104));
#24192=CARTESIAN_POINT('Ctrl Pts',(-1.10509821673782,-0.0928409665394228,
-0.204327142733962));
#24193=CARTESIAN_POINT('Ctrl Pts',(-1.10139388218929,-0.144299303100741,
-0.22376314604679));
#24194=CARTESIAN_POINT('Ctrl Pts',(-1.09728268713976,-0.177024326825049,
-0.243890930799338));
#24195=CARTESIAN_POINT('Ctrl Pts',(-1.08664560412098,-0.227269801620063,
-0.287406530683753));
#24196=CARTESIAN_POINT('Ctrl Pts',(-1.0788165083757,-0.251265615809407,
-0.316022600643821));
#24197=CARTESIAN_POINT('Ctrl Pts',(-1.06356957703048,-0.279889827963178,
-0.363699428370918));
#24198=CARTESIAN_POINT('Ctrl Pts',(-1.05494634094458,-0.290879136862659,
-0.388295406390235));
#24199=CARTESIAN_POINT('Ctrl Pts',(-1.03504317708586,-0.305251990234488,
-0.438600874831839));
#24200=CARTESIAN_POINT('Ctrl Pts',(-1.02374168767024,-0.308638795020976,
-0.46430090015576));
#24201=CARTESIAN_POINT('Ctrl Pts',(-1.00129756308006,-0.308638795020976,
-0.510906605094603));
#24202=CARTESIAN_POINT('Ctrl Pts',(-0.988250837578047,-0.305251990234488,
-0.535766169015486));
#24203=CARTESIAN_POINT('Ctrl Pts',(-0.961329858300736,-0.290879136862659,
-0.582692035672022));
#24204=CARTESIAN_POINT('Ctrl Pts',(-0.947476448101718,-0.279889827963178,
-0.604769294586516));
#24205=CARTESIAN_POINT('Ctrl Pts',(-0.919707509403859,-0.251265615809407,
-0.646415841396062));
#24206=CARTESIAN_POINT('Ctrl Pts',(-0.902215926359523,-0.227269801620064,
-0.670378702718353));
#24207=CARTESIAN_POINT('Ctrl Pts',(-0.87482617317514,-0.177024326825049,
-0.705826641853758));
#24208=CARTESIAN_POINT('Ctrl Pts',(-0.861652925570091,-0.144299303100741,
-0.721590372101268));
#24209=CARTESIAN_POINT('Ctrl Pts',(-0.848766861100456,-0.0928409665394229,
-0.736604687327351));
#24210=CARTESIAN_POINT('Ctrl Pts',(-0.84559647055299,-0.0762225747374255,
-0.740223768851063));
#24211=CARTESIAN_POINT('Ctrl Pts',(-0.843383895613249,-0.0595300000000001,
-0.742736168477219));
#24212=CARTESIAN_POINT('',(-0.536443649899847,-0.05953,-0.987512846410683));
#24213=CARTESIAN_POINT('Origin',(0.,-0.05953,0.));
#24214=CARTESIAN_POINT('',(0.0548532617164172,-0.05953,-1.12247250791415));
#24215=CARTESIAN_POINT('Ctrl Pts',(-0.536443649899848,-0.0595300000000001,
-0.987512846410683));
#24216=CARTESIAN_POINT('Ctrl Pts',(-0.533501897135712,-0.0762225747374254,
-0.989110885965947));
#24217=CARTESIAN_POINT('Ctrl Pts',(-0.529268075276156,-0.0928409665394227,
-0.991396466802469));
#24218=CARTESIAN_POINT('Ctrl Pts',(-0.511762781179147,-0.144299303100741,
-1.00061845128527));
#24219=CARTESIAN_POINT('Ctrl Pts',(-0.493462957200432,-0.177024326825049,
-1.0099536580922));
#24220=CARTESIAN_POINT('Ctrl Pts',(-0.45280897844858,-0.227269801620063,
-1.02876878445619));
#24221=CARTESIAN_POINT('Ctrl Pts',(-0.425554672694337,-0.251265615809407,
-1.04048957871266));
#24222=CARTESIAN_POINT('Ctrl Pts',(-0.3787731215897,-0.279889827963178,
-1.05829506364875));
#24223=CARTESIAN_POINT('Ctrl Pts',(-0.354166711873529,-0.290879136862659,
-1.06688848765783));
#24224=CARTESIAN_POINT('Ctrl Pts',(-0.302426893214944,-0.305251990234488,
-1.08269251410343));
#24225=CARTESIAN_POINT('Ctrl Pts',(-0.275287440920027,-0.308638795020976,
-1.0898803575765));
#24226=CARTESIAN_POINT('Ctrl Pts',(-0.224855950742601,-0.308638795020976,
-1.10139101611326));
#24227=CARTESIAN_POINT('Ctrl Pts',(-0.19728546073067,-0.305251990234488,
-1.10669035995599));
#24228=CARTESIAN_POINT('Ctrl Pts',(-0.143812384801039,-0.290879136862659,
-1.11490049012186));
#24229=CARTESIAN_POINT('Ctrl Pts',(-0.117914228755037,-0.279889827963178,
-1.1178344036749));
#24230=CARTESIAN_POINT('Ctrl Pts',(-0.0680399972366989,-0.251265615809407,
-1.12208997038458));
#24231=CARTESIAN_POINT('Ctrl Pts',(-0.0383992541984084,-0.227269801620063,
-1.12335509974011));
#24232=CARTESIAN_POINT('Ctrl Pts',(0.00639229239215326,-0.177024326825049,
-1.12404235695137));
#24233=CARTESIAN_POINT('Ctrl Pts',(0.0269302585198977,-0.144299303100741,
-1.12357162229597));
#24234=CARTESIAN_POINT('Ctrl Pts',(0.04670325263426,-0.0928409665394228,
-1.12285816383385));
#24235=CARTESIAN_POINT('Ctrl Pts',(0.0515094706813703,-0.0762225747374255,
-1.12263591311425));
#24236=CARTESIAN_POINT('Ctrl Pts',(0.0548532617164176,-0.0595300000000001,
-1.12247250791414));
#24237=CARTESIAN_POINT('',(0.437601487681057,-0.05953,-1.03511272300331));
#24238=CARTESIAN_POINT('Origin',(0.,-0.05953,0.));
#24239=CARTESIAN_POINT('',(0.911784794170997,-0.05953,-0.656964154625313));
#24240=CARTESIAN_POINT('Ctrl Pts',(0.437601487681056,-0.0595300000000001,
-1.03511272300331));
#24241=CARTESIAN_POINT('Ctrl Pts',(0.440685038163619,-0.0762225747374255,
-1.03380912944435));
#24242=CARTESIAN_POINT('Ctrl Pts',(0.445111721969657,-0.0928409665394228,
-1.03192403056628));
#24243=CARTESIAN_POINT('Ctrl Pts',(0.463236132117164,-0.144299303100741,
-1.0239876538093));
#24244=CARTESIAN_POINT('Ctrl Pts',(0.481944444320713,-0.177024326825049,
-1.01550068154148));
#24245=CARTESIAN_POINT('Ctrl Pts',(0.522002043615455,-0.227269801620064,
-0.995447160474328));
#24246=CARTESIAN_POINT('Ctrl Pts',(0.548158511259203,-0.251265615809407,
-0.981446681891443));
#24247=CARTESIAN_POINT('Ctrl Pts',(0.591247219971725,-0.279889827963178,
-0.955972930713954));
#24248=CARTESIAN_POINT('Ctrl Pts',(0.613307674922609,-0.290879136862659,
-0.942092777160053));
#24249=CARTESIAN_POINT('Ctrl Pts',(0.657923009631182,-0.305251990234487,
-0.91149460735272));
#24250=CARTESIAN_POINT('Ctrl Pts',(0.680463863683393,-0.308638795020976,
-0.894757676234429));
#24251=CARTESIAN_POINT('Ctrl Pts',(0.720906778729542,-0.308638795020976,
-0.862505527716294));
#24252=CARTESIAN_POINT('Ctrl Pts',(0.742239891936899,-0.305251990234488,
-0.844254137480381));
#24253=CARTESIAN_POINT('Ctrl Pts',(0.781998747691872,-0.290879136862659,
-0.80756613568454));
#24254=CARTESIAN_POINT('Ctrl Pts',(0.800439809856112,-0.279889827963178,
-0.789147407129765));
#24255=CARTESIAN_POINT('Ctrl Pts',(0.834863020612702,-0.251265615809407,
-0.752807465209441));
#24256=CARTESIAN_POINT('Ctrl Pts',(0.854332839576145,-0.227269801620064,
-0.73042219438957));
#24257=CARTESIAN_POINT('Ctrl Pts',(0.882797231409153,-0.177024326825049,
-0.695831250979106));
#24258=CARTESIAN_POINT('Ctrl Pts',(0.895234408667242,-0.144299303100741,
-0.679480524217551));
#24259=CARTESIAN_POINT('Ctrl Pts',(0.907004864562642,-0.0928409665394228,
-0.663576540841106));
#24260=CARTESIAN_POINT('Ctrl Pts',(0.909827729890942,-0.0762225747374256,
-0.659680317203144));
#24261=CARTESIAN_POINT('Ctrl Pts',(0.911784794170998,-0.0595300000000001,
-0.656964154625312));
#24262=CARTESIAN_POINT('',(1.08212377959455,-0.05953,-0.303251606722892));
#24263=CARTESIAN_POINT('Origin',(0.,-0.05953,0.));
#24264=CARTESIAN_POINT('',(1.08212377959455,-0.05953,0.303251606722892));
#24265=CARTESIAN_POINT('Ctrl Pts',(1.08212377959455,-0.0595300000000001,
-0.303251606722892));
#24266=CARTESIAN_POINT('Ctrl Pts',(1.0830271513892,-0.0762225747374255,
-0.300028012588062));
#24267=CARTESIAN_POINT('Ctrl Pts',(1.08431331394788,-0.0928409665394228,
-0.2953917518996));
#24268=CARTESIAN_POINT('Ctrl Pts',(1.08940878963422,-0.144299303100741,
-0.276273267473431));
#24269=CARTESIAN_POINT('Ctrl Pts',(1.09443784939331,-0.177024326825049,
-0.256354979351213));
#24270=CARTESIAN_POINT('Ctrl Pts',(1.10373487993589,-0.227269801620064,
-0.212533521233765));
#24271=CARTESIAN_POINT('Ctrl Pts',(1.10909715583869,-0.251265615809407,
-0.183354415742157));
#24272=CARTESIAN_POINT('Ctrl Pts',(1.1160463456491,-0.279889827963178,-0.133783682657561));
#24273=CARTESIAN_POINT('Ctrl Pts',(1.11894887330541,-0.290879136862659,
-0.107881990270302));
#24274=CARTESIAN_POINT('Ctrl Pts',(1.12284346704144,-0.305251990234488,
-0.0539226701638766));
#24275=CARTESIAN_POINT('Ctrl Pts',(1.123812,-0.308638795020976,-0.025864214957475));
#24276=CARTESIAN_POINT('Ctrl Pts',(1.123812,-0.308638795020976,0.025864214957475));
#24277=CARTESIAN_POINT('Ctrl Pts',(1.12284346704144,-0.305251990234488,
0.0539226701638766));
#24278=CARTESIAN_POINT('Ctrl Pts',(1.11894887330541,-0.290879136862659,
0.107881990270302));
#24279=CARTESIAN_POINT('Ctrl Pts',(1.1160463456491,-0.279889827963178,0.133783682657561));
#24280=CARTESIAN_POINT('Ctrl Pts',(1.10909715583869,-0.251265615809407,
0.183354415742157));
#24281=CARTESIAN_POINT('Ctrl Pts',(1.10373487993589,-0.227269801620064,
0.212533521233765));
#24282=CARTESIAN_POINT('Ctrl Pts',(1.09443784939331,-0.177024326825049,
0.256354979351213));
#24283=CARTESIAN_POINT('Ctrl Pts',(1.08940878963422,-0.144299303100741,
0.276273267473431));
#24284=CARTESIAN_POINT('Ctrl Pts',(1.08431331394788,-0.0928409665394228,
0.2953917518996));
#24285=CARTESIAN_POINT('Ctrl Pts',(1.0830271513892,-0.0762225747374255,
0.300028012588062));
#24286=CARTESIAN_POINT('Ctrl Pts',(1.08212377959455,-0.0595300000000001,
0.303251606722892));
#24287=CARTESIAN_POINT('Origin',(0.,-0.05953,0.));
#24288=CARTESIAN_POINT('Origin',(0.,-0.05953,0.));
#24289=CARTESIAN_POINT('',(0.0589974094846122,-0.05953,1.07456964270265));
#24290=CARTESIAN_POINT('Origin',(0.,-0.05953,0.));
#24291=CARTESIAN_POINT('Origin',(-0.244773027351946,-0.05953,1.07242070340001));
#24292=CARTESIAN_POINT('Origin',(-0.244773027351946,0.,1.07242070340001));
#24293=CARTESIAN_POINT('',(-0.519393123750572,-0.05953,0.942555777842682));
#24294=CARTESIAN_POINT('Ctrl Pts',(-0.519393123750572,-0.05953,0.942555777842682));
#24295=CARTESIAN_POINT('Ctrl Pts',(-0.513714466572041,-0.0925528133349865,
0.945684988399766));
#24296=CARTESIAN_POINT('Ctrl Pts',(-0.503136848051455,-0.124911173756694,
0.951483858396181));
#24297=CARTESIAN_POINT('Ctrl Pts',(-0.47593627990192,-0.177924977804098,
0.965323333309091));
#24298=CARTESIAN_POINT('Ctrl Pts',(-0.460931856495794,-0.199697230012983,
0.972669835243841));
#24299=CARTESIAN_POINT('Ctrl Pts',(-0.426157505475872,-0.237895043532788,
0.988400002689705));
#24300=CARTESIAN_POINT('Ctrl Pts',(-0.406380688682952,-0.254319232363049,
0.996771768218699));
#24301=CARTESIAN_POINT('Ctrl Pts',(-0.364750145543744,-0.28018331644634,
1.01272583306292));
#24302=CARTESIAN_POINT('Ctrl Pts',(-0.340838910881557,-0.29104845371857,
1.02112815447116));
#24303=CARTESIAN_POINT('Ctrl Pts',(-0.290495481564827,-0.30527573347708,
1.036574285215));
#24304=CARTESIAN_POINT('Ctrl Pts',(-0.264056468041074,-0.308638795020976,
1.04359501395068));
#24305=CARTESIAN_POINT('Ctrl Pts',(-0.214892249704082,-0.308638795020976,
1.05481642595959));
#24306=CARTESIAN_POINT('Ctrl Pts',(-0.188025341585962,-0.30527573347708,
1.05996242598502));
#24307=CARTESIAN_POINT('Ctrl Pts',(-0.135965654106109,-0.29104845371857,
1.06788913840721));
#24308=CARTESIAN_POINT('Ctrl Pts',(-0.110776745452494,-0.28018331644634,
1.07069360430242));
#24309=CARTESIAN_POINT('Ctrl Pts',(-0.0663467128214646,-0.254319232363049,
1.07438230428002));
#24310=CARTESIAN_POINT('Ctrl Pts',(-0.0448960436540983,-0.237895043532788,
1.07542044338697));
#24311=CARTESIAN_POINT('Ctrl Pts',(-0.00674037211528124,-0.199697230012983,
1.07633607767727));
#24312=CARTESIAN_POINT('Ctrl Pts',(0.00996567398334777,-0.177924977804098,
1.07622728347683));
#24313=CARTESIAN_POINT('Ctrl Pts',(0.0404772621979741,-0.124911173756694,
1.07556023164702));
#24314=CARTESIAN_POINT('Ctrl Pts',(0.0525234025782719,-0.0925528133349865,
1.07492508698591));
#24315=CARTESIAN_POINT('Ctrl Pts',(0.0589974094846124,-0.05953,1.07456964270265));
#24316=CARTESIAN_POINT('Origin',(-0.244773027351946,-0.05953,1.07242070340001));
#24317=CARTESIAN_POINT('Origin',(0.,-0.05953,0.));
#24318=CARTESIAN_POINT('',(-0.803348093619616,-0.05953,0.716109245731214));
#24319=CARTESIAN_POINT('Origin',(0.,-0.05953,0.));
#24320=CARTESIAN_POINT('Origin',(-0.991065754692661,-0.05953,0.477272113029314));
#24321=CARTESIAN_POINT('Origin',(-0.991065754692661,0.,0.477272113029314));
#24322=CARTESIAN_POINT('',(-1.06075609691358,-0.05953,0.181596019242328));
#24323=CARTESIAN_POINT('Ctrl Pts',(-1.06075609691358,-0.05953,0.181596019242328));
#24324=CARTESIAN_POINT('Ctrl Pts',(-1.05966202740332,-0.0925528133349865,
0.187986803072856));
#24325=CARTESIAN_POINT('Ctrl Pts',(-1.05760072925372,-0.124911173756694,
0.199872254546857));
#24326=CARTESIAN_POINT('Ctrl Pts',(-1.05146158959546,-0.177924977804098,
0.22976728653846));
#24327=CARTESIAN_POINT('Ctrl Pts',(-1.04785021111757,-0.199697230012983,
0.246078686169301));
#24328=CARTESIAN_POINT('Ctrl Pts',(-1.03846709802406,-0.237895043532788,
0.283073967563097));
#24329=CARTESIAN_POINT('Ctrl Pts',(-1.03268176429485,-0.254319232363049,
0.303755815985685));
#24330=CARTESIAN_POINT('Ctrl Pts',(-1.01919893537026,-0.28018331644634,
0.346251081972725));
#24331=CARTESIAN_POINT('Ctrl Pts',(-1.01085972381132,-0.29104845371857,
0.370184399726282));
#24332=CARTESIAN_POINT('Ctrl Pts',(-0.99154738033959,-0.30527573347708,
0.419174982698463));
#24333=CARTESIAN_POINT('Ctrl Pts',(-0.980551951791748,-0.308638795020976,
0.444223188605045));
#24334=CARTESIAN_POINT('Ctrl Pts',(-0.958671816228589,-0.308638795020976,
0.489657758261848));
#24335=CARTESIAN_POINT('Ctrl Pts',(-0.945943877838127,-0.30527573347708,
0.51387163140139));
#24336=CARTESIAN_POINT('Ctrl Pts',(-0.91968254693063,-0.29104845371857,
0.559515758398093));
#24337=CARTESIAN_POINT('Ctrl Pts',(-0.906170138993533,-0.28018331644634,
0.580957796077825));
#24338=CARTESIAN_POINT('Ctrl Pts',(-0.8813524085237,-0.254319232363049,
0.617994461173994));
#24339=CARTESIAN_POINT('Ctrl Pts',(-0.868789784891799,-0.237895043532788,
0.635412538795143));
#24340=CARTESIAN_POINT('Ctrl Pts',(-0.845715984518854,-0.199697230012983,
0.66581473268113));
#24341=CARTESIAN_POINT('Ctrl Pts',(-0.835214876415962,-0.177924977804098,
0.678808213394124));
#24342=CARTESIAN_POINT('Ctrl Pts',(-0.815669690204649,-0.124911173756694,
0.702247233627224));
#24343=CARTESIAN_POINT('Ctrl Pts',(-0.807662468433796,-0.0925528133349865,
0.711269279199861));
#24344=CARTESIAN_POINT('Ctrl Pts',(-0.803348093619616,-0.05953,0.716109245731214));
#24345=CARTESIAN_POINT('Origin',(-0.991065754692661,-0.05953,0.477272113029314));
#24346=CARTESIAN_POINT('Origin',(0.,-0.05953,0.));
#24347=CARTESIAN_POINT('',(-1.076188,-0.05953,1.31795018948079E-16));
#24348=CARTESIAN_POINT('Origin',(0.,-0.05953,0.));
#24349=CARTESIAN_POINT('',(-1.06075609691358,-0.05953,-0.181596019242328));
#24350=CARTESIAN_POINT('Origin',(0.,-0.05953,0.));
#24351=CARTESIAN_POINT('Origin',(-0.991065754692661,-0.05953,-0.477272113029314));
#24352=CARTESIAN_POINT('Origin',(-0.991065754692661,0.,-0.477272113029314));
#24353=CARTESIAN_POINT('',(-0.803348093619616,-0.05953,-0.716109245731215));
#24354=CARTESIAN_POINT('Ctrl Pts',(-0.803348093619616,-0.05953,-0.716109245731215));
#24355=CARTESIAN_POINT('Ctrl Pts',(-0.807662468433795,-0.0925528133349865,
-0.711269279199862));
#24356=CARTESIAN_POINT('Ctrl Pts',(-0.815669690204649,-0.124911173756694,
-0.702247233627224));
#24357=CARTESIAN_POINT('Ctrl Pts',(-0.835214876415962,-0.177924977804098,
-0.678808213394124));
#24358=CARTESIAN_POINT('Ctrl Pts',(-0.845715984518854,-0.199697230012983,
-0.66581473268113));
#24359=CARTESIAN_POINT('Ctrl Pts',(-0.868789784891799,-0.237895043532788,
-0.635412538795143));
#24360=CARTESIAN_POINT('Ctrl Pts',(-0.8813524085237,-0.254319232363049,
-0.617994461173994));
#24361=CARTESIAN_POINT('Ctrl Pts',(-0.906170138993533,-0.28018331644634,
-0.580957796077826));
#24362=CARTESIAN_POINT('Ctrl Pts',(-0.91968254693063,-0.29104845371857,
-0.559515758398093));
#24363=CARTESIAN_POINT('Ctrl Pts',(-0.945943877838127,-0.30527573347708,
-0.51387163140139));
#24364=CARTESIAN_POINT('Ctrl Pts',(-0.958671816228589,-0.308638795020976,
-0.489657758261848));
#24365=CARTESIAN_POINT('Ctrl Pts',(-0.980551951791748,-0.308638795020976,
-0.444223188605045));
#24366=CARTESIAN_POINT('Ctrl Pts',(-0.99154738033959,-0.30527573347708,
-0.419174982698463));
#24367=CARTESIAN_POINT('Ctrl Pts',(-1.01085972381132,-0.29104845371857,
-0.370184399726282));
#24368=CARTESIAN_POINT('Ctrl Pts',(-1.01919893537026,-0.28018331644634,
-0.346251081972725));
#24369=CARTESIAN_POINT('Ctrl Pts',(-1.03268176429485,-0.254319232363049,
-0.303755815985685));
#24370=CARTESIAN_POINT('Ctrl Pts',(-1.03846709802406,-0.237895043532788,
-0.283073967563097));
#24371=CARTESIAN_POINT('Ctrl Pts',(-1.04785021111757,-0.199697230012983,
-0.246078686169302));
#24372=CARTESIAN_POINT('Ctrl Pts',(-1.05146158959546,-0.177924977804098,
-0.229767286538461));
#24373=CARTESIAN_POINT('Ctrl Pts',(-1.05760072925372,-0.124911173756694,
-0.199872254546858));
#24374=CARTESIAN_POINT('Ctrl Pts',(-1.05966202740332,-0.0925528133349864,
-0.187986803072857));
#24375=CARTESIAN_POINT('Ctrl Pts',(-1.06075609691358,-0.05953,-0.181596019242328));
#24376=CARTESIAN_POINT('Origin',(-0.991065754692661,-0.05953,-0.477272113029314));
#24377=CARTESIAN_POINT('Origin',(0.,-0.05953,0.));
#24378=CARTESIAN_POINT('',(-0.519393123750572,-0.05953,-0.942555777842682));
#24379=CARTESIAN_POINT('Origin',(0.,-0.05953,0.));
#24380=CARTESIAN_POINT('Origin',(-0.244773027351946,-0.05953,-1.07242070340001));
#24381=CARTESIAN_POINT('Origin',(-0.244773027351946,0.,-1.07242070340001));
#24382=CARTESIAN_POINT('',(0.0589974094846125,-0.05953,-1.07456964270265));
#24383=CARTESIAN_POINT('Ctrl Pts',(0.0589974094846127,-0.05953,-1.07456964270265));
#24384=CARTESIAN_POINT('Ctrl Pts',(0.0525234025782722,-0.0925528133349865,
-1.07492508698591));
#24385=CARTESIAN_POINT('Ctrl Pts',(0.0404772621979744,-0.124911173756694,
-1.07556023164702));
#24386=CARTESIAN_POINT('Ctrl Pts',(0.0099656739833481,-0.177924977804098,
-1.07622728347683));
#24387=CARTESIAN_POINT('Ctrl Pts',(-0.00674037211528096,-0.199697230012983,
-1.07633607767727));
#24388=CARTESIAN_POINT('Ctrl Pts',(-0.044896043654098,-0.237895043532788,
-1.07542044338697));
#24389=CARTESIAN_POINT('Ctrl Pts',(-0.0663467128214644,-0.254319232363049,
-1.07438230428002));
#24390=CARTESIAN_POINT('Ctrl Pts',(-0.110776745452493,-0.28018331644634,
-1.07069360430242));
#24391=CARTESIAN_POINT('Ctrl Pts',(-0.135965654106109,-0.29104845371857,
-1.06788913840721));
#24392=CARTESIAN_POINT('Ctrl Pts',(-0.188025341585962,-0.30527573347708,
-1.05996242598502));
#24393=CARTESIAN_POINT('Ctrl Pts',(-0.214892249704082,-0.308638795020976,
-1.05481642595959));
#24394=CARTESIAN_POINT('Ctrl Pts',(-0.264056468041074,-0.308638795020976,
-1.04359501395068));
#24395=CARTESIAN_POINT('Ctrl Pts',(-0.290495481564827,-0.30527573347708,
-1.036574285215));
#24396=CARTESIAN_POINT('Ctrl Pts',(-0.340838910881557,-0.291048453718569,
-1.02112815447116));
#24397=CARTESIAN_POINT('Ctrl Pts',(-0.364750145543744,-0.28018331644634,
-1.01272583306292));
#24398=CARTESIAN_POINT('Ctrl Pts',(-0.406380688682952,-0.254319232363049,
-0.996771768218699));
#24399=CARTESIAN_POINT('Ctrl Pts',(-0.426157505475872,-0.237895043532788,
-0.988400002689705));
#24400=CARTESIAN_POINT('Ctrl Pts',(-0.460931856495794,-0.199697230012983,
-0.972669835243841));
#24401=CARTESIAN_POINT('Ctrl Pts',(-0.475936279901919,-0.177924977804098,
-0.965323333309091));
#24402=CARTESIAN_POINT('Ctrl Pts',(-0.503136848051454,-0.124911173756694,
-0.951483858396181));
#24403=CARTESIAN_POINT('Ctrl Pts',(-0.513714466572041,-0.0925528133349865,
-0.945684988399766));
#24404=CARTESIAN_POINT('Ctrl Pts',(-0.519393123750572,-0.05953,-0.942555777842682));
#24405=CARTESIAN_POINT('Origin',(-0.244773027351946,-0.05953,-1.07242070340001));
#24406=CARTESIAN_POINT('Origin',(0.,-0.05953,0.));
#24407=CARTESIAN_POINT('',(0.413083465285518,-0.05953,-0.993751811093549));
#24408=CARTESIAN_POINT('Origin',(0.,-0.05953,0.));
#24409=CARTESIAN_POINT('Origin',(0.685838782044607,-0.05953,-0.860014630714833));
#24410=CARTESIAN_POINT('Origin',(0.685838782044607,0.,-0.860014630714833));
#24411=CARTESIAN_POINT('',(0.876916659919095,-0.05953,-0.623857181492959));
#24412=CARTESIAN_POINT('Ctrl Pts',(0.876916659919095,-0.05953,-0.623857181492958));
#24413=CARTESIAN_POINT('Ctrl Pts',(0.873158080166742,-0.0925528133349865,
-0.62914037979579));
#24414=CARTESIAN_POINT('Ctrl Pts',(0.866144010579847,-0.124911173756694,
-0.638954437806245));
#24415=CARTESIAN_POINT('Ctrl Pts',(0.847641868610495,-0.177924977804098,
-0.663225258065736));
#24416=CARTESIAN_POINT('Ctrl Pts',(0.837310877969633,-0.199697230012983,
-0.676354402927683));
#24417=CARTESIAN_POINT('Ctrl Pts',(0.81280533416753,-0.237895043532788,
-0.705614819529209));
#24418=CARTESIAN_POINT('Ctrl Pts',(0.798619410861634,-0.254319232363049,
-0.721738358858166));
#24419=CARTESIAN_POINT('Ctrl Pts',(0.768033796848072,-0.28018331644634,
-0.754175290318038));
#24420=CARTESIAN_POINT('Ctrl Pts',(0.750136149454208,-0.29104845371857,
-0.772120216227122));
#24421=CARTESIAN_POINT('Ctrl Pts',(0.711480111898423,-0.30527573347708,
-0.807879894508811));
#24422=CARTESIAN_POINT('Ctrl Pts',(0.690705563850638,-0.308638795020976,
-0.825676810575913));
#24423=CARTESIAN_POINT('Ctrl Pts',(0.651278921914856,-0.308638795020976,
-0.857118508332695));
#24424=CARTESIAN_POINT('Ctrl Pts',(0.629305439856167,-0.30527573347708,
-0.873412008702649));
#24425=CARTESIAN_POINT('Ctrl Pts',(0.585840553788742,-0.29104845371857,
-0.903141581680914));
#24426=CARTESIAN_POINT('Ctrl Pts',(0.564362943424239,-0.28018331644634,
-0.916597376014514));
#24427=CARTESIAN_POINT('Ctrl Pts',(0.525933334162556,-0.254319232363049,
-0.939198248544427));
#24428=CARTESIAN_POINT('Ctrl Pts',(0.507057380724533,-0.237895043532788,
-0.949440676105255));
#24429=CARTESIAN_POINT('Ctrl Pts',(0.473077587363686,-0.199697230012983,
-0.966820759530997));
#24430=CARTESIAN_POINT('Ctrl Pts',(0.457978755888596,-0.177924977804098,
-0.973971221090534));
#24431=CARTESIAN_POINT('Ctrl Pts',(0.430199341854858,-0.124911173756694,
-0.986608710139579));
#24432=CARTESIAN_POINT('Ctrl Pts',(0.419070565453384,-0.0925528133349865,
-0.991263089003441));
#24433=CARTESIAN_POINT('Ctrl Pts',(0.413083465285518,-0.05953,-0.993751811093549));
#24434=CARTESIAN_POINT('Origin',(0.685838782044607,-0.05953,-0.860014630714833));
#24435=CARTESIAN_POINT('Origin',(0.,-0.208355,0.));
#24436=CARTESIAN_POINT('',(-1.076188,-0.35718,1.31795018948079E-16));
#24437=CARTESIAN_POINT('Origin',(0.,-0.35718,0.));
#24438=CARTESIAN_POINT('',(-1.076188,-0.208355,1.31795018948079E-16));
#24439=CARTESIAN_POINT('',(1.03449977959455,-0.05953,0.296632461748266));
#24440=CARTESIAN_POINT('Origin',(0.,-0.05953,0.));
#24441=CARTESIAN_POINT('',(1.03449977959455,-0.05953,-0.296632461748266));
#24442=CARTESIAN_POINT('Ctrl Pts',(1.03449977959455,-0.05953,0.296632461748267));
#24443=CARTESIAN_POINT('Ctrl Pts',(1.03628691421076,-0.0925528133349865,
0.290399865505497));
#24444=CARTESIAN_POINT('Ctrl Pts',(1.03958665287714,-0.124911173756694,
0.278797079997872));
#24445=CARTESIAN_POINT('Ctrl Pts',(1.0470264474309,-0.177924977804098,0.249198913998601));
#24446=CARTESIAN_POINT('Ctrl Pts',(1.05084995891418,-0.199697230012983,
0.232935932341942));
#24447=CARTESIAN_POINT('Ctrl Pts',(1.05844771715377,-0.237895043532788,
0.195533155353269));
#24448=CARTESIAN_POINT('Ctrl Pts',(1.06220882929878,-0.254319232363049,
0.17438929156337));
#24449=CARTESIAN_POINT('Ctrl Pts',(1.06849922508772,-0.28018331644634,0.130252399648131));
#24450=CARTESIAN_POINT('Ctrl Pts',(1.07137013248666,-0.29104845371857,0.105070977154072));
#24451=CARTESIAN_POINT('Ctrl Pts',(1.07522652957392,-0.30527573347708,0.0525526752791107));
#24452=CARTESIAN_POINT('Ctrl Pts',(1.076188,-0.308638795020976,0.025214283908933));
#24453=CARTESIAN_POINT('Ctrl Pts',(1.076188,-0.308638795020976,-0.025214283908933));
#24454=CARTESIAN_POINT('Ctrl Pts',(1.07522652957392,-0.30527573347708,-0.0525526752791107));
#24455=CARTESIAN_POINT('Ctrl Pts',(1.07137013248666,-0.29104845371857,-0.105070977154072));
#24456=CARTESIAN_POINT('Ctrl Pts',(1.06849922508772,-0.28018331644634,-0.130252399648131));
#24457=CARTESIAN_POINT('Ctrl Pts',(1.06220882929878,-0.254319232363049,
-0.17438929156337));
#24458=CARTESIAN_POINT('Ctrl Pts',(1.05844771715377,-0.237895043532788,
-0.195533155353269));
#24459=CARTESIAN_POINT('Ctrl Pts',(1.05084995891418,-0.199697230012983,
-0.232935932341942));
#24460=CARTESIAN_POINT('Ctrl Pts',(1.0470264474309,-0.177924977804098,-0.249198913998601));
#24461=CARTESIAN_POINT('Ctrl Pts',(1.03958665287714,-0.124911173756694,
-0.278797079997872));
#24462=CARTESIAN_POINT('Ctrl Pts',(1.03628691421076,-0.0925528133349865,
-0.290399865505497));
#24463=CARTESIAN_POINT('Ctrl Pts',(1.03449977959455,-0.05953,-0.296632461748267));
#24464=CARTESIAN_POINT('Origin',(0.,-0.05953,0.));
#24465=CARTESIAN_POINT('Origin',(0.,-0.05953,0.));
#24466=CARTESIAN_POINT('Origin',(1.1,-0.05953,0.));
#24467=CARTESIAN_POINT('Origin',(1.1,0.,0.));
#24468=CARTESIAN_POINT('Origin',(1.1,-0.05953,0.));
#24469=CARTESIAN_POINT('Origin',(0.,-0.35718,0.));
#24470=CARTESIAN_POINT('Origin',(0.,-0.05953,0.));
#62628=UNCERTAINTY_MEASURE_WITH_UNIT(LENGTH_MEASURE(0.001),#62759,
'DISTANCE_ACCURACY_VALUE',
'Maximum model space distance between geometric entities at asserted c
onnectivities');
#62684=UNCERTAINTY_MEASURE_WITH_UNIT(LENGTH_MEASURE(0.001),#62759,
'DISTANCE_ACCURACY_VALUE',
'Maximum model space distance between geometric entities at asserted c
onnectivities');
#62702=(
GEOMETRIC_REPRESENTATION_CONTEXT(3)
GLOBAL_UNCERTAINTY_ASSIGNED_CONTEXT((#62628))
GLOBAL_UNIT_ASSIGNED_CONTEXT((#62759,#62761,#62762))
REPRESENTATION_CONTEXT('','3D')
);
#62758=(
GEOMETRIC_REPRESENTATION_CONTEXT(3)
GLOBAL_UNCERTAINTY_ASSIGNED_CONTEXT((#62684))
GLOBAL_UNIT_ASSIGNED_CONTEXT((#62759,#62761,#62762))
REPRESENTATION_CONTEXT('','3D')
);
#62759=(
LENGTH_UNIT()
NAMED_UNIT(*)
SI_UNIT(.CENTI.,.METRE.)
);
#62761=(
NAMED_UNIT(*)
PLANE_ANGLE_UNIT()
SI_UNIT($,.RADIAN.)
);
#62762=(
NAMED_UNIT(*)
SI_UNIT($,.STERADIAN.)
SOLID_ANGLE_UNIT()
);
#62780=SHAPE_DEFINITION_REPRESENTATION(#62853,#63048);
#62853=PRODUCT_DEFINITION_SHAPE('',$,#63122);
#63048=SHAPE_REPRESENTATION('',(#17540),#62702);
#63104=PRODUCT_DEFINITION_CONTEXT('part definition',#63325,'design');
#63122=PRODUCT_DEFINITION('Cage','Cage',#63195,#63104);
#63195=PRODUCT_DEFINITION_FORMATION('',$,#63344);
#63325=APPLICATION_CONTEXT(
'Core Data for Automotive Mechanical Design Process');
#63326=PRODUCT_CONTEXT('part definition',#63325,'mechanical');
#63344=PRODUCT('Cage','Cage','Cage',(#63326));
#63456=COLOUR_RGB('Grey',0.48,0.52,0.57);
#63457=FILL_AREA_STYLE_COLOUR('',#63456);
#63458=FILL_AREA_STYLE('',(#63457));
#63459=SURFACE_STYLE_FILL_AREA(#63458);
#63460=SURFACE_SIDE_STYLE('',(#63459));
#63461=SURFACE_STYLE_USAGE(.BOTH.,#63460);
#63462=PRESENTATION_STYLE_ASSIGNMENT((#63461));
ENDSEC;
END-ISO-10303-21;
